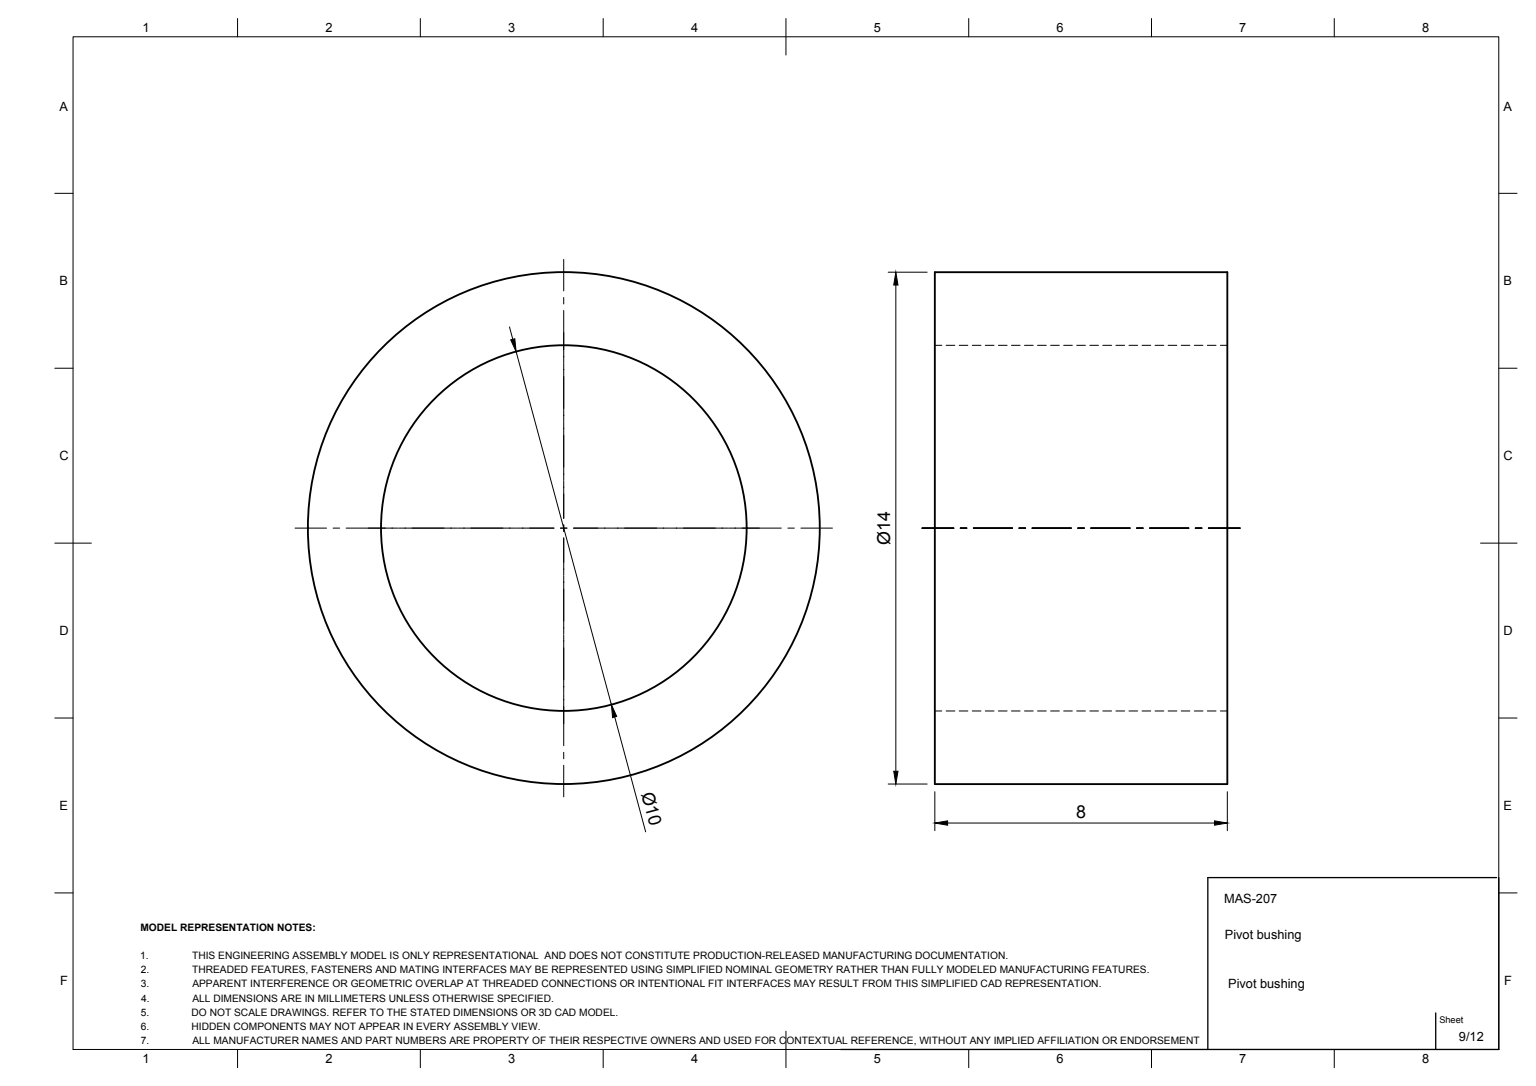
ISO-10303-21;
HEADER;
/* Generated by software containing ST-Developer
 * from STEP Tools, Inc. (www.steptools.com) 
 */

FILE_DESCRIPTION(
/* description */ ('Independent six-slot Geneva indexer. Center distance100, drive radius
50, 60degree indexing per input revolution with120degree engagement an
d240degree dwell. Native machined concave locking faces and relieved d
isk; replaceable retained drive pin; keyed output shaft. Geometry traj
ectory checks use calculated indexing positions, not a contact-dynamic
s simulation. No load or production rating assigned.'),
/* implementation_level */ '2;1');

FILE_NAME(
/* name */ 'Pivot bushing.step',
/* time_stamp */ '2026-11-09T17:53:22-08:00',
/* author */ (''),
/* organization */ (''),
/* preprocessor_version */ 'ST-DEVELOPER v20.2',
/* originating_system */ 'Autodesk Translation Framework v15.17.0.0',
/* authorisation */ '');

FILE_SCHEMA (('AUTOMOTIVE_DESIGN { 1 0 10303 214 3 1 1 }'));
ENDSEC;

DATA;
#10=MECHANICAL_DESIGN_GEOMETRIC_PRESENTATION_REPRESENTATION('',(#107),#4149);
#85=SHAPE_REPRESENTATION_RELATIONSHIP('SRR','None',#4202,#96);
#96=ADVANCED_BREP_SHAPE_REPRESENTATION('',(#118),#4144);
#107=STYLED_ITEM('',(#4265),#118);
#118=MANIFOLD_SOLID_BREP('Body1',#2301);
#153=FACE_BOUND('',#521,.T.);
#154=FACE_BOUND('',#523,.T.);
#226=PLANE('',#2660);
#227=PLANE('',#2661);
#352=FACE_OUTER_BOUND('',#518,.T.);
#353=FACE_OUTER_BOUND('',#519,.T.);
#354=FACE_OUTER_BOUND('',#520,.T.);
#355=FACE_OUTER_BOUND('',#522,.T.);
#518=EDGE_LOOP('',(#2028,#2029,#2030,#2031));
#519=EDGE_LOOP('',(#2032,#2033,#2034,#2035));
#520=EDGE_LOOP('',(#2036));
#521=EDGE_LOOP('',(#2037));
#522=EDGE_LOOP('',(#2038));
#523=EDGE_LOOP('',(#2039));
#704=LINE('',#4025,#876);
#705=LINE('',#4031,#877);
#876=VECTOR('',#3329,5.);
#877=VECTOR('',#3336,7.);
#996=CIRCLE('',#2655,5.);
#997=CIRCLE('',#2656,5.);
#998=CIRCLE('',#2658,7.);
#999=CIRCLE('',#2659,7.);
#1188=VERTEX_POINT('',#4022);
#1189=VERTEX_POINT('',#4024);
#1190=VERTEX_POINT('',#4028);
#1191=VERTEX_POINT('',#4030);
#1472=EDGE_CURVE('',#1188,#1188,#996,.T.);
#1473=EDGE_CURVE('',#1188,#1189,#704,.T.);
#1474=EDGE_CURVE('',#1189,#1189,#997,.T.);
#1475=EDGE_CURVE('',#1190,#1190,#998,.T.);
#1476=EDGE_CURVE('',#1190,#1191,#705,.T.);
#1477=EDGE_CURVE('',#1191,#1191,#999,.T.);
#2028=ORIENTED_EDGE('',*,*,#1472,.F.);
#2029=ORIENTED_EDGE('',*,*,#1473,.T.);
#2030=ORIENTED_EDGE('',*,*,#1474,.T.);
#2031=ORIENTED_EDGE('',*,*,#1473,.F.);
#2032=ORIENTED_EDGE('',*,*,#1475,.F.);
#2033=ORIENTED_EDGE('',*,*,#1476,.T.);
#2034=ORIENTED_EDGE('',*,*,#1477,.T.);
#2035=ORIENTED_EDGE('',*,*,#1476,.F.);
#2036=ORIENTED_EDGE('',*,*,#1475,.T.);
#2037=ORIENTED_EDGE('',*,*,#1472,.T.);
#2038=ORIENTED_EDGE('',*,*,#1477,.F.);
#2039=ORIENTED_EDGE('',*,*,#1474,.F.);
#2149=CYLINDRICAL_SURFACE('',#2654,5.);
#2150=CYLINDRICAL_SURFACE('',#2657,7.);
#2273=ADVANCED_FACE('',(#352),#2149,.F.);
#2274=ADVANCED_FACE('',(#353),#2150,.T.);
#2275=ADVANCED_FACE('',(#354,#153),#226,.T.);
#2276=ADVANCED_FACE('',(#355,#154),#227,.F.);
#2301=CLOSED_SHELL('',(#2273,#2274,#2275,#2276));
#2653=AXIS2_PLACEMENT_3D('',#4020,#3323,#3324);
#2654=AXIS2_PLACEMENT_3D('',#4021,#3325,#3326);
#2655=AXIS2_PLACEMENT_3D('',#4023,#3327,#3328);
#2656=AXIS2_PLACEMENT_3D('',#4026,#3330,#3331);
#2657=AXIS2_PLACEMENT_3D('',#4027,#3332,#3333);
#2658=AXIS2_PLACEMENT_3D('',#4029,#3334,#3335);
#2659=AXIS2_PLACEMENT_3D('',#4032,#3337,#3338);
#2660=AXIS2_PLACEMENT_3D('',#4033,#3339,#3340);
#2661=AXIS2_PLACEMENT_3D('',#4034,#3341,#3342);
#3323=DIRECTION('axis',(0.,0.,1.));
#3324=DIRECTION('refdir',(1.,0.,0.));
#3325=DIRECTION('center_axis',(0.,0.,1.));
#3326=DIRECTION('ref_axis',(1.,0.,0.));
#3327=DIRECTION('center_axis',(0.,0.,-1.));
#3328=DIRECTION('ref_axis',(1.,0.,0.));
#3329=DIRECTION('',(0.,0.,-1.));
#3330=DIRECTION('center_axis',(0.,0.,-1.));
#3331=DIRECTION('ref_axis',(1.,0.,0.));
#3332=DIRECTION('center_axis',(0.,0.,1.));
#3333=DIRECTION('ref_axis',(1.,0.,0.));
#3334=DIRECTION('center_axis',(0.,0.,1.));
#3335=DIRECTION('ref_axis',(1.,0.,0.));
#3336=DIRECTION('',(0.,0.,-1.));
#3337=DIRECTION('center_axis',(0.,0.,1.));
#3338=DIRECTION('ref_axis',(1.,0.,0.));
#3339=DIRECTION('center_axis',(0.,0.,1.));
#3340=DIRECTION('ref_axis',(1.,0.,0.));
#3341=DIRECTION('center_axis',(0.,0.,1.));
#3342=DIRECTION('ref_axis',(1.,0.,0.));
#4020=CARTESIAN_POINT('',(0.,0.,0.));
#4021=CARTESIAN_POINT('Origin',(0.,0.,0.));
#4022=CARTESIAN_POINT('',(-5.,-6.12323399573677E-16,8.));
#4023=CARTESIAN_POINT('Origin',(0.,0.,8.));
#4024=CARTESIAN_POINT('',(-5.,-6.12323399573677E-16,0.));
#4025=CARTESIAN_POINT('',(-5.,-6.12323399573677E-16,0.));
#4026=CARTESIAN_POINT('Origin',(0.,0.,0.));
#4027=CARTESIAN_POINT('Origin',(0.,0.,0.));
#4028=CARTESIAN_POINT('',(-7.,-8.57252759403147E-16,8.));
#4029=CARTESIAN_POINT('Origin',(0.,0.,8.));
#4030=CARTESIAN_POINT('',(-7.,-8.57252759403147E-16,0.));
#4031=CARTESIAN_POINT('',(-7.,-8.57252759403147E-16,0.));
#4032=CARTESIAN_POINT('Origin',(0.,0.,0.));
#4033=CARTESIAN_POINT('Origin',(0.,0.,8.));
#4034=CARTESIAN_POINT('Origin',(0.,0.,0.));
#4131=UNCERTAINTY_MEASURE_WITH_UNIT(LENGTH_MEASURE(0.01),#4150,
'DISTANCE_ACCURACY_VALUE',
'Maximum model space distance between geometric entities at asserted c
onnectivities');
#4136=UNCERTAINTY_MEASURE_WITH_UNIT(LENGTH_MEASURE(0.01),#4150,
'DISTANCE_ACCURACY_VALUE',
'Maximum model space distance between geometric entities at asserted c
onnectivities');
#4144=(
GEOMETRIC_REPRESENTATION_CONTEXT(3)
GLOBAL_UNCERTAINTY_ASSIGNED_CONTEXT((#4131))
GLOBAL_UNIT_ASSIGNED_CONTEXT((#4150,#4152,#4153))
REPRESENTATION_CONTEXT('','3D')
);
#4149=(
GEOMETRIC_REPRESENTATION_CONTEXT(3)
GLOBAL_UNCERTAINTY_ASSIGNED_CONTEXT((#4136))
GLOBAL_UNIT_ASSIGNED_CONTEXT((#4150,#4152,#4153))
REPRESENTATION_CONTEXT('','3D')
);
#4150=(
LENGTH_UNIT()
NAMED_UNIT(*)
SI_UNIT(.MILLI.,.METRE.)
);
#4152=(
NAMED_UNIT(*)
PLANE_ANGLE_UNIT()
SI_UNIT($,.RADIAN.)
);
#4153=(
NAMED_UNIT(*)
SI_UNIT($,.STERADIAN.)
SOLID_ANGLE_UNIT()
);
#4161=SHAPE_DEFINITION_REPRESENTATION(#4173,#4202);
#4173=PRODUCT_DEFINITION_SHAPE('',$,#4215);
#4202=SHAPE_REPRESENTATION('',(#2653),#4144);
#4207=PRODUCT_DEFINITION_CONTEXT('part definition',#4245,'design');
#4215=PRODUCT_DEFINITION('Pivot bushing','Pivot bushing',#4227,#4207);
#4227=PRODUCT_DEFINITION_FORMATION('',$,#4254);
#4245=APPLICATION_CONTEXT(
'Core Data for Automotive Mechanical Design Process');
#4246=PRODUCT_CONTEXT('part definition',#4245,'mechanical');
#4254=PRODUCT('Pivot bushing','Pivot bushing',$,(#4246));
#4265=PRESENTATION_STYLE_ASSIGNMENT((#4275));
#4275=SURFACE_STYLE_USAGE(.BOTH.,#4285);
#4285=SURFACE_SIDE_STYLE('',(#4295));
#4295=SURFACE_STYLE_FILL_AREA(#4305);
#4305=FILL_AREA_STYLE('Bearing light gray',(#4315));
#4315=FILL_AREA_STYLE_COLOUR('Bearing light gray',#4325);
#4325=COLOUR_RGB('Bearing light gray',0.725490196078431,0.752941176470588,
0.792156862745098);
ENDSEC;
END-ISO-10303-21;
